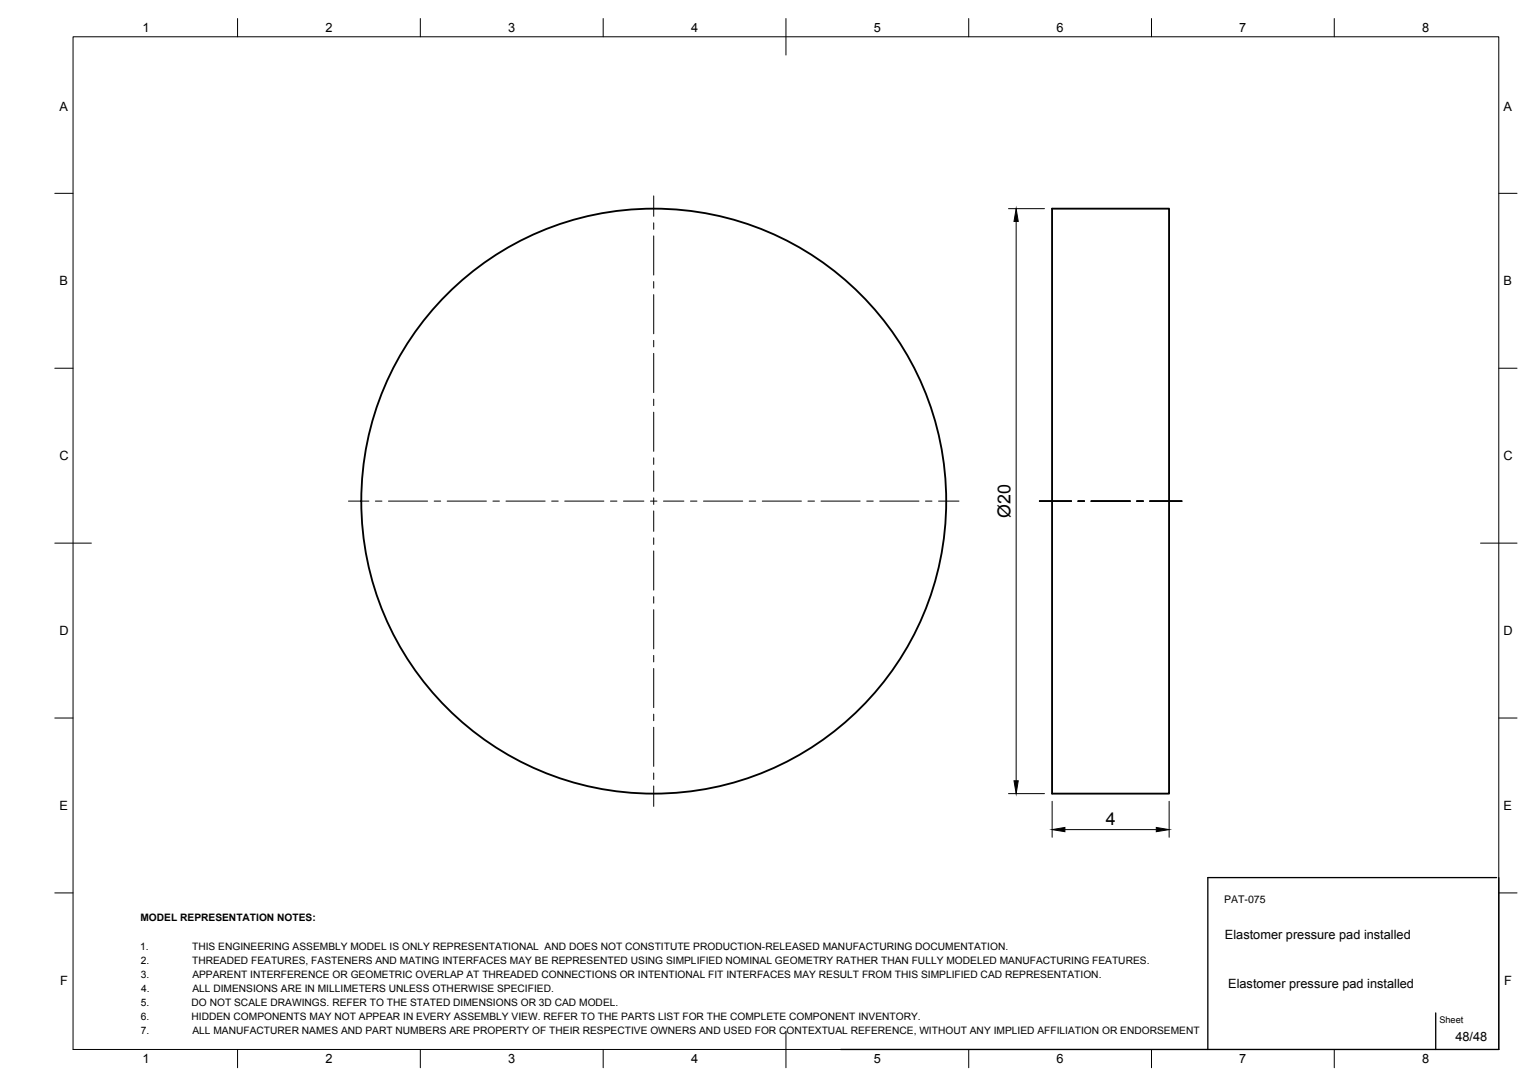
ISO-10303-21;
HEADER;
/* Generated by software containing ST-Developer
 * from STEP Tools, Inc. (www.steptools.com) 
 */

FILE_DESCRIPTION(
/* description */ ('Over-Centre Plunger Toggle Clamp on Slotted Fixture Frame'),
/* implementation_level */ '2;1');

FILE_NAME(
/* name */ 
'Elastomer pressure pad installed.step',
/* time_stamp */ '2026-10-28T03:23:24-07:00',
/* author */ (''),
/* organization */ (''),
/* preprocessor_version */ 'ST-DEVELOPER v20.2',
/* originating_system */ 'Autodesk Translation Framework v15.17.0.0',
/* authorisation */ '');

FILE_SCHEMA (('AUTOMOTIVE_DESIGN { 1 0 10303 214 3 1 1 }'));
ENDSEC;

DATA;
#10=MECHANICAL_DESIGN_GEOMETRIC_PRESENTATION_REPRESENTATION('',(#562),#15212);
#469=SHAPE_REPRESENTATION_RELATIONSHIP('SRR','None',#15448,#511);
#511=ADVANCED_BREP_SHAPE_REPRESENTATION('',(#609),#15210);
#562=STYLED_ITEM('',(#15733),#609);
#609=MANIFOLD_SOLID_BREP('Body1',#8298);
#1076=PLANE('',#9727);
#1077=PLANE('',#9728);
#1558=FACE_OUTER_BOUND('',#2215,.T.);
#1559=FACE_OUTER_BOUND('',#2216,.T.);
#1560=FACE_OUTER_BOUND('',#2217,.T.);
#2215=EDGE_LOOP('',(#7561,#7562,#7563,#7564));
#2216=EDGE_LOOP('',(#7565));
#2217=EDGE_LOOP('',(#7566));
#2839=LINE('',#15047,#3469);
#3469=VECTOR('',#12288,1.);
#3853=CIRCLE('',#9725,1.);
#3854=CIRCLE('',#9726,1.);
#4527=VERTEX_POINT('',#15044);
#4528=VERTEX_POINT('',#15046);
#5541=EDGE_CURVE('',#4527,#4527,#3853,.T.);
#5542=EDGE_CURVE('',#4527,#4528,#2839,.T.);
#5543=EDGE_CURVE('',#4528,#4528,#3854,.T.);
#7561=ORIENTED_EDGE('',*,*,#5541,.F.);
#7562=ORIENTED_EDGE('',*,*,#5542,.T.);
#7563=ORIENTED_EDGE('',*,*,#5543,.T.);
#7564=ORIENTED_EDGE('',*,*,#5542,.F.);
#7565=ORIENTED_EDGE('',*,*,#5541,.T.);
#7566=ORIENTED_EDGE('',*,*,#5543,.F.);
#7757=CYLINDRICAL_SURFACE('',#9724,1.);
#8230=ADVANCED_FACE('',(#1558),#7757,.T.);
#8231=ADVANCED_FACE('',(#1559),#1076,.T.);
#8232=ADVANCED_FACE('',(#1560),#1077,.F.);
#8298=CLOSED_SHELL('',(#8230,#8231,#8232));
#9723=AXIS2_PLACEMENT_3D('',#15042,#12282,#12283);
#9724=AXIS2_PLACEMENT_3D('',#15043,#12284,#12285);
#9725=AXIS2_PLACEMENT_3D('',#15045,#12286,#12287);
#9726=AXIS2_PLACEMENT_3D('',#15048,#12289,#12290);
#9727=AXIS2_PLACEMENT_3D('',#15049,#12291,#12292);
#9728=AXIS2_PLACEMENT_3D('',#15050,#12293,#12294);
#12282=DIRECTION('axis',(0.,0.,1.));
#12283=DIRECTION('refdir',(1.,0.,0.));
#12284=DIRECTION('center_axis',(0.,0.,1.));
#12285=DIRECTION('ref_axis',(1.,0.,0.));
#12286=DIRECTION('center_axis',(0.,0.,1.));
#12287=DIRECTION('ref_axis',(1.,0.,0.));
#12288=DIRECTION('',(0.,0.,-1.));
#12289=DIRECTION('center_axis',(0.,0.,1.));
#12290=DIRECTION('ref_axis',(1.,0.,0.));
#12291=DIRECTION('center_axis',(0.,0.,1.));
#12292=DIRECTION('ref_axis',(1.,0.,0.));
#12293=DIRECTION('center_axis',(0.,0.,1.));
#12294=DIRECTION('ref_axis',(1.,0.,0.));
#15042=CARTESIAN_POINT('',(0.,0.,0.));
#15043=CARTESIAN_POINT('Origin',(0.,0.,3.));
#15044=CARTESIAN_POINT('',(-1.,-1.22464679914735E-16,3.4));
#15045=CARTESIAN_POINT('Origin',(0.,0.,3.4));
#15046=CARTESIAN_POINT('',(-1.,-1.22464679914735E-16,3.));
#15047=CARTESIAN_POINT('',(-1.,-1.22464679914735E-16,3.));
#15048=CARTESIAN_POINT('Origin',(0.,0.,3.));
#15049=CARTESIAN_POINT('Origin',(0.,0.,3.4));
#15050=CARTESIAN_POINT('Origin',(0.,0.,3.));
#15160=UNCERTAINTY_MEASURE_WITH_UNIT(LENGTH_MEASURE(0.001),#15213,
'DISTANCE_ACCURACY_VALUE',
'Maximum model space distance between geometric entities at asserted c
onnectivities');
#15162=UNCERTAINTY_MEASURE_WITH_UNIT(LENGTH_MEASURE(0.001),#15213,
'DISTANCE_ACCURACY_VALUE',
'Maximum model space distance between geometric entities at asserted c
onnectivities');
#15210=(
GEOMETRIC_REPRESENTATION_CONTEXT(3)
GLOBAL_UNCERTAINTY_ASSIGNED_CONTEXT((#15160))
GLOBAL_UNIT_ASSIGNED_CONTEXT((#15213,#15215,#15216))
REPRESENTATION_CONTEXT('','3D')
);
#15212=(
GEOMETRIC_REPRESENTATION_CONTEXT(3)
GLOBAL_UNCERTAINTY_ASSIGNED_CONTEXT((#15162))
GLOBAL_UNIT_ASSIGNED_CONTEXT((#15213,#15215,#15216))
REPRESENTATION_CONTEXT('','3D')
);
#15213=(
LENGTH_UNIT()
NAMED_UNIT(*)
SI_UNIT(.CENTI.,.METRE.)
);
#15215=(
NAMED_UNIT(*)
PLANE_ANGLE_UNIT()
SI_UNIT($,.RADIAN.)
);
#15216=(
NAMED_UNIT(*)
SI_UNIT($,.STERADIAN.)
SOLID_ANGLE_UNIT()
);
#15264=SHAPE_DEFINITION_REPRESENTATION(#15391,#15448);
#15391=PRODUCT_DEFINITION_SHAPE('',$,#15498);
#15448=SHAPE_REPRESENTATION('',(#9723),#15210);
#15450=PRODUCT_DEFINITION_CONTEXT('part definition',#15599,'design');
#15498=PRODUCT_DEFINITION('Elastomer pressure pad installed',
'Elastomer pressure pad installed',#15547,#15450);
#15547=PRODUCT_DEFINITION_FORMATION('',$,#15648);
#15599=APPLICATION_CONTEXT(
'Core Data for Automotive Mechanical Design Process');
#15600=PRODUCT_CONTEXT('part definition',#15599,'mechanical');
#15648=PRODUCT('Elastomer pressure pad installed',
'Elastomer pressure pad installed','Elastomer pressure pad installed',(#15600));
#15727=COLOUR_RGB('Off White',0.89,0.88,0.83);
#15728=FILL_AREA_STYLE_COLOUR('',#15727);
#15729=FILL_AREA_STYLE('',(#15728));
#15730=SURFACE_STYLE_FILL_AREA(#15729);
#15731=SURFACE_SIDE_STYLE('',(#15730));
#15732=SURFACE_STYLE_USAGE(.BOTH.,#15731);
#15733=PRESENTATION_STYLE_ASSIGNMENT((#15732));
ENDSEC;
END-ISO-10303-21;
